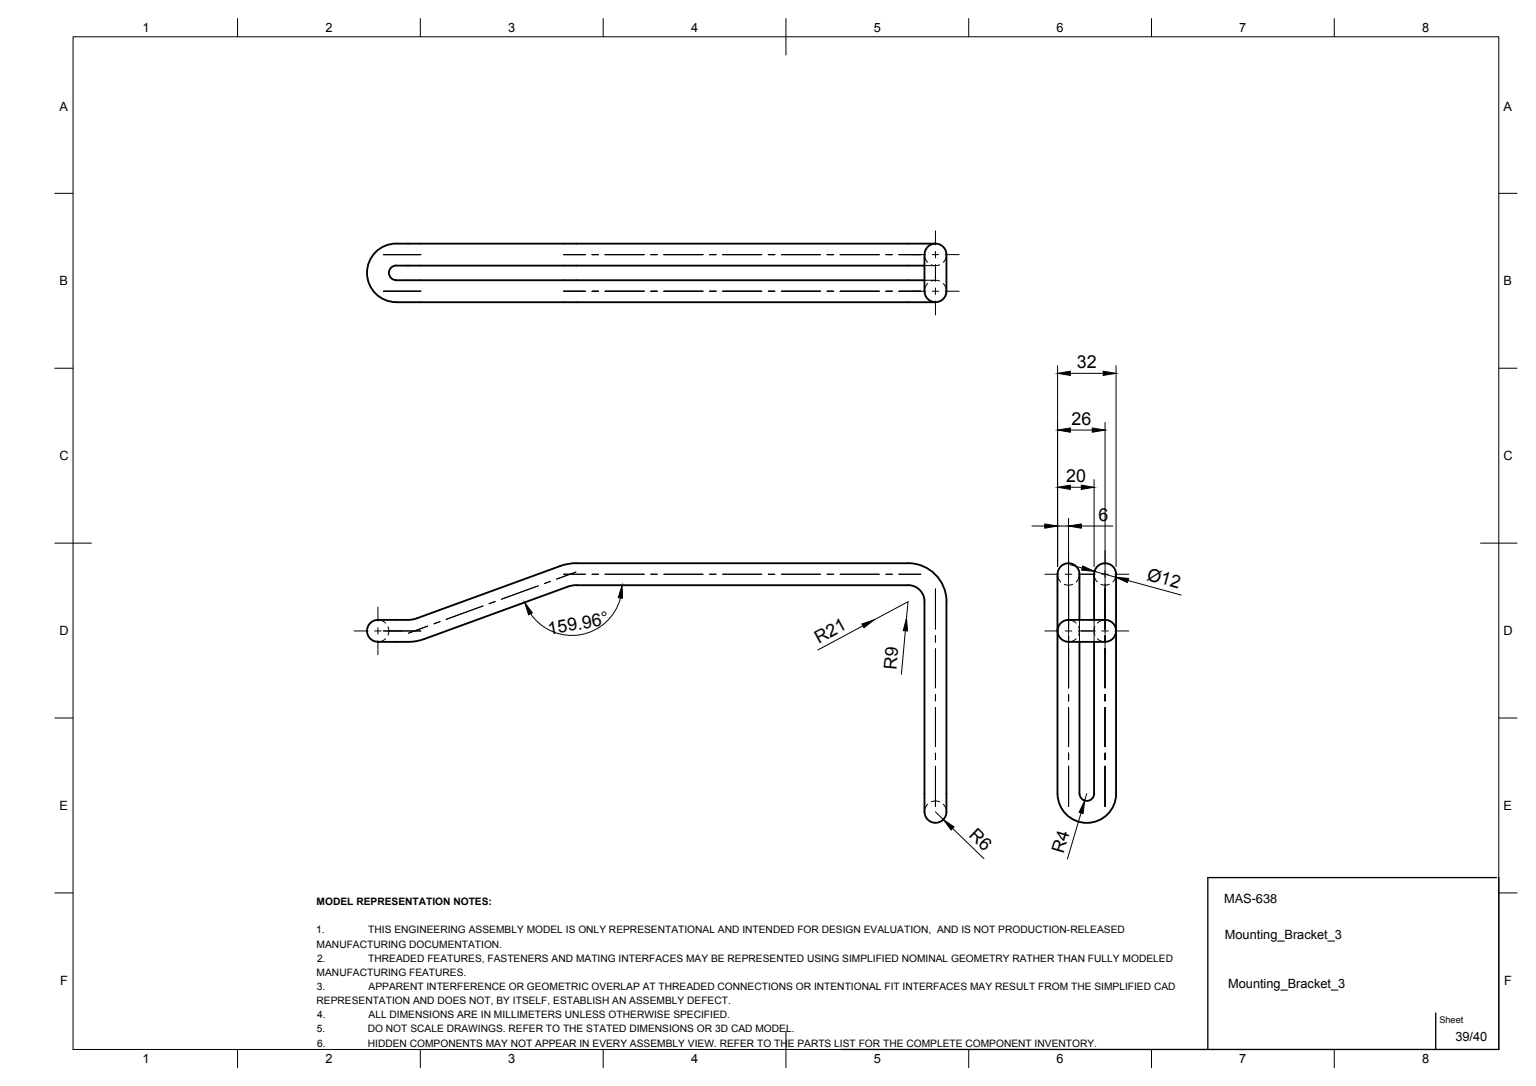
ISO-10303-21;
HEADER;
FILE_DESCRIPTION((''),'2;1');
FILE_NAME('Mounting_Bracket_3.step','2026-10-09T12:00:21-07:00',(''),(''),'','','');
FILE_SCHEMA (('AUTOMOTIVE_DESIGN { 1 0 10303 214 3 1 1 }'));
ENDSEC;
DATA;
#10=MECHANICAL_DESIGN_GEOMETRIC_PRESENTATION_REPRESENTATION('',(#434),#10334);
#176=CYLINDRICAL_SURFACE('',#4377,0.600000000000001) ;
#177=CYLINDRICAL_SURFACE('',#4378,0.600000000000001) ;
#178=CYLINDRICAL_SURFACE('',#4379,0.599999999999997) ;
#179=CYLINDRICAL_SURFACE('',#4380,0.600000000000001) ;
#180=CYLINDRICAL_SURFACE('',#4381,0.600000000000001) ;
#181=CYLINDRICAL_SURFACE('',#4382,0.600000000000001) ;
#182=CYLINDRICAL_SURFACE('',#4383,0.599999999999997) ;
#183=CYLINDRICAL_SURFACE('',#4384,0.600000000000001) ;
#362=SHAPE_REPRESENTATION_RELATIONSHIP('SRR','None',#10480,#394) ;
#394=ADVANCED_BREP_SHAPE_REPRESENTATION('',(#466),#10332) ;
#434=STYLED_ITEM('',(#10631),#466) ;
#466=MANIFOLD_SOLID_BREP('Body1',#3588) ;
#674=LINE('',#10153,#832) ;
#675=LINE('',#10155,#833) ;
#676=LINE('',#10157,#834) ;
#677=LINE('',#10159,#835) ;
#678=LINE('',#10161,#836) ;
#679=LINE('',#10163,#837) ;
#680=LINE('',#10165,#838) ;
#681=LINE('',#10167,#839) ;
#832=VECTOR('',#5456,0.600000000000001) ;
#833=VECTOR('',#5459,0.600000000000001) ;
#834=VECTOR('',#5462,0.599999999999997) ;
#835=VECTOR('',#5465,0.600000000000001) ;
#836=VECTOR('',#5468,0.600000000000001) ;
#837=VECTOR('',#5471,0.600000000000001) ;
#838=VECTOR('',#5474,0.599999999999997) ;
#839=VECTOR('',#5477,0.600000000000001) ;
#1018=FACE_OUTER_BOUND('',#1226,.T.) ;
#1019=FACE_OUTER_BOUND('',#1227,.T.) ;
#1020=FACE_OUTER_BOUND('',#1228,.T.) ;
#1021=FACE_OUTER_BOUND('',#1229,.T.) ;
#1022=FACE_OUTER_BOUND('',#1230,.T.) ;
#1023=FACE_OUTER_BOUND('',#1231,.T.) ;
#1024=FACE_OUTER_BOUND('',#1232,.T.) ;
#1025=FACE_OUTER_BOUND('',#1233,.T.) ;
#1026=FACE_OUTER_BOUND('',#1234,.T.) ;
#1027=FACE_OUTER_BOUND('',#1235,.T.) ;
#1028=FACE_OUTER_BOUND('',#1236,.T.) ;
#1029=FACE_OUTER_BOUND('',#1237,.T.) ;
#1030=FACE_OUTER_BOUND('',#1238,.T.) ;
#1031=FACE_OUTER_BOUND('',#1239,.T.) ;
#1032=FACE_OUTER_BOUND('',#1240,.T.) ;
#1033=FACE_OUTER_BOUND('',#1241,.T.) ;
#1226=EDGE_LOOP('',(#3133,#3134,#3135,#3136,#3137)) ;
#1227=EDGE_LOOP('',(#3138,#3139,#3140,#3141)) ;
#1228=EDGE_LOOP('',(#3142,#3143,#3144,#3145,#3146,#3147)) ;
#1229=EDGE_LOOP('',(#3148,#3149,#3150,#3151,#3152,#3153)) ;
#1230=EDGE_LOOP('',(#3154,#3155,#3156,#3157,#3158,#3159)) ;
#1231=EDGE_LOOP('',(#3160,#3161,#3162,#3163,#3164)) ;
#1232=EDGE_LOOP('',(#3165,#3166,#3167,#3168)) ;
#1233=EDGE_LOOP('',(#3169,#3170,#3171,#3172,#3173,#3174)) ;
#1234=EDGE_LOOP('',(#3175,#3176,#3177,#3178,#3179,#3180)) ;
#1235=EDGE_LOOP('',(#3181,#3182,#3183,#3184)) ;
#1236=EDGE_LOOP('',(#3185,#3186,#3187,#3188,#3189)) ;
#1237=EDGE_LOOP('',(#3190,#3191,#3192,#3193,#3194,#3195)) ;
#1238=EDGE_LOOP('',(#3196,#3197,#3198,#3199,#3200,#3201)) ;
#1239=EDGE_LOOP('',(#3202,#3203,#3204,#3205)) ;
#1240=EDGE_LOOP('',(#3206,#3207,#3208,#3209,#3210)) ;
#1241=EDGE_LOOP('',(#3211,#3212,#3213,#3214,#3215,#3216)) ;
#1431=CIRCLE('',#4336,0.600000000000001) ;
#1432=CIRCLE('',#4337,0.9) ;
#1433=CIRCLE('',#4338,0.600000000000001) ;
#1434=CIRCLE('',#4339,0.600000000000001) ;
#1435=CIRCLE('',#4341,0.600000000000001) ;
#1436=CIRCLE('',#4342,1.4) ;
#1437=CIRCLE('',#4343,0.600000000000001) ;
#1438=CIRCLE('',#4345,0.600000000000001) ;
#1439=CIRCLE('',#4346,0.600000000000001) ;
#1440=CIRCLE('',#4347,1.4) ;
#1441=CIRCLE('',#4348,0.600000000000001) ;
#1442=CIRCLE('',#4349,0.600000000000001) ;
#1443=CIRCLE('',#4351,0.600000000000001) ;
#1444=CIRCLE('',#4352,0.400000000000006) ;
#1445=CIRCLE('',#4353,0.600000000000001) ;
#1446=CIRCLE('',#4354,0.600000000000001) ;
#1447=CIRCLE('',#4355,0.600000000000001) ;
#1448=CIRCLE('',#4357,0.600000000000001) ;
#1449=CIRCLE('',#4358,0.600000000000001) ;
#1450=CIRCLE('',#4359,0.400000000000006) ;
#1451=CIRCLE('',#4360,0.600000000000001) ;
#1452=CIRCLE('',#4361,0.600000000000001) ;
#1453=CIRCLE('',#4363,0.600000000000001) ;
#1454=CIRCLE('',#4364,0.600000000000001) ;
#1455=CIRCLE('',#4365,0.9) ;
#1456=CIRCLE('',#4366,0.600000000000001) ;
#1457=CIRCLE('',#4368,0.600000000000001) ;
#1458=CIRCLE('',#4369,1.4) ;
#1459=CIRCLE('',#4370,0.600000000000001) ;
#1460=CIRCLE('',#4372,0.600000000000001) ;
#1461=CIRCLE('',#4373,0.600000000000001) ;
#1462=CIRCLE('',#4374,1.4) ;
#1463=CIRCLE('',#4375,0.600000000000001) ;
#1464=CIRCLE('',#4376,0.600000000000001) ;
#1758=VERTEX_POINT('',#10085) ;
#1759=VERTEX_POINT('',#10087) ;
#1760=VERTEX_POINT('',#10089) ;
#1761=VERTEX_POINT('',#10093) ;
#1762=VERTEX_POINT('',#10095) ;
#1763=VERTEX_POINT('',#10099) ;
#1764=VERTEX_POINT('',#10100) ;
#1765=VERTEX_POINT('',#10103) ;
#1766=VERTEX_POINT('',#10105) ;
#1767=VERTEX_POINT('',#10109) ;
#1768=VERTEX_POINT('',#10110) ;
#1769=VERTEX_POINT('',#10112) ;
#1770=VERTEX_POINT('',#10114) ;
#1771=VERTEX_POINT('',#10119) ;
#1772=VERTEX_POINT('',#10120) ;
#1773=VERTEX_POINT('',#10123) ;
#1774=VERTEX_POINT('',#10125) ;
#1775=VERTEX_POINT('',#10129) ;
#1776=VERTEX_POINT('',#10130) ;
#1777=VERTEX_POINT('',#10133) ;
#1778=VERTEX_POINT('',#10137) ;
#1779=VERTEX_POINT('',#10139) ;
#1780=VERTEX_POINT('',#10143) ;
#1781=VERTEX_POINT('',#10144) ;
#1782=VERTEX_POINT('',#10147) ;
#1783=VERTEX_POINT('',#10149) ;
#2223=EDGE_CURVE('',#1758,#1758,#1431,.T.) ;
#2224=EDGE_CURVE('',#1758,#1759,#1432,.T.) ;
#2225=EDGE_CURVE('',#1759,#1760,#1433,.T.) ;
#2226=EDGE_CURVE('',#1760,#1759,#1434,.T.) ;
#2227=EDGE_CURVE('',#1761,#1761,#1435,.T.) ;
#2228=EDGE_CURVE('',#1761,#1762,#1436,.T.) ;
#2229=EDGE_CURVE('',#1762,#1762,#1437,.T.) ;
#2230=EDGE_CURVE('',#1763,#1764,#1438,.T.) ;
#2231=EDGE_CURVE('',#1764,#1763,#1439,.T.) ;
#2232=EDGE_CURVE('',#1764,#1765,#1440,.T.) ;
#2233=EDGE_CURVE('',#1765,#1766,#1441,.T.) ;
#2234=EDGE_CURVE('',#1766,#1765,#1442,.T.) ;
#2235=EDGE_CURVE('',#1767,#1768,#1443,.T.) ;
#2236=EDGE_CURVE('',#1768,#1769,#1444,.T.) ;
#2237=EDGE_CURVE('',#1770,#1769,#1445,.T.) ;
#2238=EDGE_CURVE('',#1769,#1770,#1446,.T.) ;
#2239=EDGE_CURVE('',#1768,#1767,#1447,.T.) ;
#2240=EDGE_CURVE('',#1771,#1772,#1448,.T.) ;
#2241=EDGE_CURVE('',#1772,#1771,#1449,.T.) ;
#2242=EDGE_CURVE('',#1772,#1773,#1450,.T.) ;
#2243=EDGE_CURVE('',#1773,#1774,#1451,.T.) ;
#2244=EDGE_CURVE('',#1774,#1773,#1452,.T.) ;
#2245=EDGE_CURVE('',#1775,#1776,#1453,.T.) ;
#2246=EDGE_CURVE('',#1776,#1775,#1454,.T.) ;
#2247=EDGE_CURVE('',#1776,#1777,#1455,.T.) ;
#2248=EDGE_CURVE('',#1777,#1777,#1456,.T.) ;
#2249=EDGE_CURVE('',#1778,#1778,#1457,.T.) ;
#2250=EDGE_CURVE('',#1778,#1779,#1458,.T.) ;
#2251=EDGE_CURVE('',#1779,#1779,#1459,.T.) ;
#2252=EDGE_CURVE('',#1780,#1781,#1460,.T.) ;
#2253=EDGE_CURVE('',#1781,#1780,#1461,.T.) ;
#2254=EDGE_CURVE('',#1781,#1782,#1462,.T.) ;
#2255=EDGE_CURVE('',#1782,#1783,#1463,.T.) ;
#2256=EDGE_CURVE('',#1783,#1782,#1464,.T.) ;
#2257=EDGE_CURVE('',#1771,#1760,#674,.T.) ;
#2258=EDGE_CURVE('',#1758,#1762,#675,.T.) ;
#2259=EDGE_CURVE('',#1761,#1766,#676,.T.) ;
#2260=EDGE_CURVE('',#1763,#1767,#677,.T.) ;
#2261=EDGE_CURVE('',#1774,#1775,#678,.T.) ;
#2262=EDGE_CURVE('',#1777,#1778,#679,.T.) ;
#2263=EDGE_CURVE('',#1779,#1780,#680,.T.) ;
#2264=EDGE_CURVE('',#1783,#1770,#681,.T.) ;
#3133=ORIENTED_EDGE('',*,*,#2223,.F.) ;
#3134=ORIENTED_EDGE('',*,*,#2224,.T.) ;
#3135=ORIENTED_EDGE('',*,*,#2225,.T.) ;
#3136=ORIENTED_EDGE('',*,*,#2226,.T.) ;
#3137=ORIENTED_EDGE('',*,*,#2224,.F.) ;
#3138=ORIENTED_EDGE('',*,*,#2227,.F.) ;
#3139=ORIENTED_EDGE('',*,*,#2228,.T.) ;
#3140=ORIENTED_EDGE('',*,*,#2229,.T.) ;
#3141=ORIENTED_EDGE('',*,*,#2228,.F.) ;
#3142=ORIENTED_EDGE('',*,*,#2230,.F.) ;
#3143=ORIENTED_EDGE('',*,*,#2231,.F.) ;
#3144=ORIENTED_EDGE('',*,*,#2232,.T.) ;
#3145=ORIENTED_EDGE('',*,*,#2233,.T.) ;
#3146=ORIENTED_EDGE('',*,*,#2234,.T.) ;
#3147=ORIENTED_EDGE('',*,*,#2232,.F.) ;
#3148=ORIENTED_EDGE('',*,*,#2235,.T.) ;
#3149=ORIENTED_EDGE('',*,*,#2236,.T.) ;
#3150=ORIENTED_EDGE('',*,*,#2237,.F.) ;
#3151=ORIENTED_EDGE('',*,*,#2238,.F.) ;
#3152=ORIENTED_EDGE('',*,*,#2236,.F.) ;
#3153=ORIENTED_EDGE('',*,*,#2239,.T.) ;
#3154=ORIENTED_EDGE('',*,*,#2240,.F.) ;
#3155=ORIENTED_EDGE('',*,*,#2241,.F.) ;
#3156=ORIENTED_EDGE('',*,*,#2242,.T.) ;
#3157=ORIENTED_EDGE('',*,*,#2243,.T.) ;
#3158=ORIENTED_EDGE('',*,*,#2244,.T.) ;
#3159=ORIENTED_EDGE('',*,*,#2242,.F.) ;
#3160=ORIENTED_EDGE('',*,*,#2245,.F.) ;
#3161=ORIENTED_EDGE('',*,*,#2246,.F.) ;
#3162=ORIENTED_EDGE('',*,*,#2247,.T.) ;
#3163=ORIENTED_EDGE('',*,*,#2248,.T.) ;
#3164=ORIENTED_EDGE('',*,*,#2247,.F.) ;
#3165=ORIENTED_EDGE('',*,*,#2249,.F.) ;
#3166=ORIENTED_EDGE('',*,*,#2250,.T.) ;
#3167=ORIENTED_EDGE('',*,*,#2251,.T.) ;
#3168=ORIENTED_EDGE('',*,*,#2250,.F.) ;
#3169=ORIENTED_EDGE('',*,*,#2252,.F.) ;
#3170=ORIENTED_EDGE('',*,*,#2253,.F.) ;
#3171=ORIENTED_EDGE('',*,*,#2254,.T.) ;
#3172=ORIENTED_EDGE('',*,*,#2255,.T.) ;
#3173=ORIENTED_EDGE('',*,*,#2256,.T.) ;
#3174=ORIENTED_EDGE('',*,*,#2254,.F.) ;
#3175=ORIENTED_EDGE('',*,*,#2240,.T.) ;
#3176=ORIENTED_EDGE('',*,*,#2241,.T.) ;
#3177=ORIENTED_EDGE('',*,*,#2257,.T.) ;
#3178=ORIENTED_EDGE('',*,*,#2225,.F.) ;
#3179=ORIENTED_EDGE('',*,*,#2226,.F.) ;
#3180=ORIENTED_EDGE('',*,*,#2257,.F.) ;
#3181=ORIENTED_EDGE('',*,*,#2223,.T.) ;
#3182=ORIENTED_EDGE('',*,*,#2258,.T.) ;
#3183=ORIENTED_EDGE('',*,*,#2229,.F.) ;
#3184=ORIENTED_EDGE('',*,*,#2258,.F.) ;
#3185=ORIENTED_EDGE('',*,*,#2227,.T.) ;
#3186=ORIENTED_EDGE('',*,*,#2259,.T.) ;
#3187=ORIENTED_EDGE('',*,*,#2233,.F.) ;
#3188=ORIENTED_EDGE('',*,*,#2234,.F.) ;
#3189=ORIENTED_EDGE('',*,*,#2259,.F.) ;
#3190=ORIENTED_EDGE('',*,*,#2230,.T.) ;
#3191=ORIENTED_EDGE('',*,*,#2231,.T.) ;
#3192=ORIENTED_EDGE('',*,*,#2260,.T.) ;
#3193=ORIENTED_EDGE('',*,*,#2239,.F.) ;
#3194=ORIENTED_EDGE('',*,*,#2235,.F.) ;
#3195=ORIENTED_EDGE('',*,*,#2260,.F.) ;
#3196=ORIENTED_EDGE('',*,*,#2244,.F.) ;
#3197=ORIENTED_EDGE('',*,*,#2261,.T.) ;
#3198=ORIENTED_EDGE('',*,*,#2245,.T.) ;
#3199=ORIENTED_EDGE('',*,*,#2246,.T.) ;
#3200=ORIENTED_EDGE('',*,*,#2261,.F.) ;
#3201=ORIENTED_EDGE('',*,*,#2243,.F.) ;
#3202=ORIENTED_EDGE('',*,*,#2248,.F.) ;
#3203=ORIENTED_EDGE('',*,*,#2262,.T.) ;
#3204=ORIENTED_EDGE('',*,*,#2249,.T.) ;
#3205=ORIENTED_EDGE('',*,*,#2262,.F.) ;
#3206=ORIENTED_EDGE('',*,*,#2251,.F.) ;
#3207=ORIENTED_EDGE('',*,*,#2263,.T.) ;
#3208=ORIENTED_EDGE('',*,*,#2252,.T.) ;
#3209=ORIENTED_EDGE('',*,*,#2253,.T.) ;
#3210=ORIENTED_EDGE('',*,*,#2263,.F.) ;
#3211=ORIENTED_EDGE('',*,*,#2256,.F.) ;
#3212=ORIENTED_EDGE('',*,*,#2264,.T.) ;
#3213=ORIENTED_EDGE('',*,*,#2237,.T.) ;
#3214=ORIENTED_EDGE('',*,*,#2238,.T.) ;
#3215=ORIENTED_EDGE('',*,*,#2264,.F.) ;
#3216=ORIENTED_EDGE('',*,*,#2255,.F.) ;
#3343=TOROIDAL_SURFACE('',#4335,1.5,0.6) ;
#3344=TOROIDAL_SURFACE('',#4340,2.,0.6) ;
#3345=TOROIDAL_SURFACE('',#4344,2.,0.6) ;
#3346=TOROIDAL_SURFACE('',#4350,1.,0.6) ;
#3347=TOROIDAL_SURFACE('',#4356,1.,0.599999999999999) ;
#3348=TOROIDAL_SURFACE('',#4362,1.5,0.6) ;
#3349=TOROIDAL_SURFACE('',#4367,2.,0.6) ;
#3350=TOROIDAL_SURFACE('',#4371,2.,0.6) ;
#3526=ADVANCED_FACE('',(#1018),#3343,.T.) ;
#3527=ADVANCED_FACE('',(#1019),#3344,.T.) ;
#3528=ADVANCED_FACE('',(#1020),#3345,.T.) ;
#3529=ADVANCED_FACE('',(#1021),#3346,.T.) ;
#3530=ADVANCED_FACE('',(#1022),#3347,.T.) ;
#3531=ADVANCED_FACE('',(#1023),#3348,.T.) ;
#3532=ADVANCED_FACE('',(#1024),#3349,.T.) ;
#3533=ADVANCED_FACE('',(#1025),#3350,.T.) ;
#3534=ADVANCED_FACE('',(#1026),#176,.T.) ;
#3535=ADVANCED_FACE('',(#1027),#177,.T.) ;
#3536=ADVANCED_FACE('',(#1028),#178,.T.) ;
#3537=ADVANCED_FACE('',(#1029),#179,.T.) ;
#3538=ADVANCED_FACE('',(#1030),#180,.T.) ;
#3539=ADVANCED_FACE('',(#1031),#181,.T.) ;
#3540=ADVANCED_FACE('',(#1032),#182,.T.) ;
#3541=ADVANCED_FACE('',(#1033),#183,.T.) ;
#3588=CLOSED_SHELL('',(#3526,#3527,#3528,#3529,#3530,#3531,#3532,#3533,
#3534,#3535,#3536,#3537,#3538,#3539,#3540,#3541)) ;
#4334=AXIS2_PLACEMENT_3D('',#10083,#5368,#5369) ;
#4335=AXIS2_PLACEMENT_3D('',#10084,#5370,#5371) ;
#4336=AXIS2_PLACEMENT_3D('',#10086,#5372,#5373) ;
#4337=AXIS2_PLACEMENT_3D('',#10088,#5374,#5375) ;
#4338=AXIS2_PLACEMENT_3D('',#10090,#5376,#5377) ;
#4339=AXIS2_PLACEMENT_3D('',#10091,#5378,#5379) ;
#4340=AXIS2_PLACEMENT_3D('',#10092,#5380,#5381) ;
#4341=AXIS2_PLACEMENT_3D('',#10094,#5382,#5383) ;
#4342=AXIS2_PLACEMENT_3D('',#10096,#5384,#5385) ;
#4343=AXIS2_PLACEMENT_3D('',#10097,#5386,#5387) ;
#4344=AXIS2_PLACEMENT_3D('',#10098,#5388,#5389) ;
#4345=AXIS2_PLACEMENT_3D('',#10101,#5390,#5391) ;
#4346=AXIS2_PLACEMENT_3D('',#10102,#5392,#5393) ;
#4347=AXIS2_PLACEMENT_3D('',#10104,#5394,#5395) ;
#4348=AXIS2_PLACEMENT_3D('',#10106,#5396,#5397) ;
#4349=AXIS2_PLACEMENT_3D('',#10107,#5398,#5399) ;
#4350=AXIS2_PLACEMENT_3D('',#10108,#5400,#5401) ;
#4351=AXIS2_PLACEMENT_3D('',#10111,#5402,#5403) ;
#4352=AXIS2_PLACEMENT_3D('',#10113,#5404,#5405) ;
#4353=AXIS2_PLACEMENT_3D('',#10115,#5406,#5407) ;
#4354=AXIS2_PLACEMENT_3D('',#10116,#5408,#5409) ;
#4355=AXIS2_PLACEMENT_3D('',#10117,#5410,#5411) ;
#4356=AXIS2_PLACEMENT_3D('',#10118,#5412,#5413) ;
#4357=AXIS2_PLACEMENT_3D('',#10121,#5414,#5415) ;
#4358=AXIS2_PLACEMENT_3D('',#10122,#5416,#5417) ;
#4359=AXIS2_PLACEMENT_3D('',#10124,#5418,#5419) ;
#4360=AXIS2_PLACEMENT_3D('',#10126,#5420,#5421) ;
#4361=AXIS2_PLACEMENT_3D('',#10127,#5422,#5423) ;
#4362=AXIS2_PLACEMENT_3D('',#10128,#5424,#5425) ;
#4363=AXIS2_PLACEMENT_3D('',#10131,#5426,#5427) ;
#4364=AXIS2_PLACEMENT_3D('',#10132,#5428,#5429) ;
#4365=AXIS2_PLACEMENT_3D('',#10134,#5430,#5431) ;
#4366=AXIS2_PLACEMENT_3D('',#10135,#5432,#5433) ;
#4367=AXIS2_PLACEMENT_3D('',#10136,#5434,#5435) ;
#4368=AXIS2_PLACEMENT_3D('',#10138,#5436,#5437) ;
#4369=AXIS2_PLACEMENT_3D('',#10140,#5438,#5439) ;
#4370=AXIS2_PLACEMENT_3D('',#10141,#5440,#5441) ;
#4371=AXIS2_PLACEMENT_3D('',#10142,#5442,#5443) ;
#4372=AXIS2_PLACEMENT_3D('',#10145,#5444,#5445) ;
#4373=AXIS2_PLACEMENT_3D('',#10146,#5446,#5447) ;
#4374=AXIS2_PLACEMENT_3D('',#10148,#5448,#5449) ;
#4375=AXIS2_PLACEMENT_3D('',#10150,#5450,#5451) ;
#4376=AXIS2_PLACEMENT_3D('',#10151,#5452,#5453) ;
#4377=AXIS2_PLACEMENT_3D('',#10152,#5454,#5455) ;
#4378=AXIS2_PLACEMENT_3D('',#10154,#5457,#5458) ;
#4379=AXIS2_PLACEMENT_3D('',#10156,#5460,#5461) ;
#4380=AXIS2_PLACEMENT_3D('',#10158,#5463,#5464) ;
#4381=AXIS2_PLACEMENT_3D('',#10160,#5466,#5467) ;
#4382=AXIS2_PLACEMENT_3D('',#10162,#5469,#5470) ;
#4383=AXIS2_PLACEMENT_3D('',#10164,#5472,#5473) ;
#4384=AXIS2_PLACEMENT_3D('',#10166,#5475,#5476) ;
#5368=DIRECTION('axis',(0.,0.,1.)) ;
#5369=DIRECTION('refdir',(1.,0.,0.)) ;
#5370=DIRECTION('center_axis',(6.88094734232038E-15,0.,-1.)) ;
#5371=DIRECTION('ref_axis',(1.,0.,6.76707367390572E-15)) ;
#5372=DIRECTION('center_axis',(1.,0.,6.88094734232038E-15)) ;
#5373=DIRECTION('ref_axis',(6.88094734232038E-15,0.,-1.)) ;
#5374=DIRECTION('center_axis',(-6.88094734232038E-15,0.,1.)) ;
#5375=DIRECTION('ref_axis',(1.,0.,6.88094734232038E-15)) ;
#5376=DIRECTION('center_axis',(0.,1.,0.)) ;
#5377=DIRECTION('ref_axis',(4.62592926927148E-15,0.,-1.)) ;
#5378=DIRECTION('center_axis',(0.,1.,0.)) ;
#5379=DIRECTION('ref_axis',(4.62592926927148E-15,0.,-1.)) ;
#5380=DIRECTION('center_axis',(6.88094734232038E-15,0.,-1.)) ;
#5381=DIRECTION('ref_axis',(1.,0.,5.46571335200077E-15)) ;
#5382=DIRECTION('center_axis',(0.93947030108257,-0.342630345100702,6.46444567142303E-15)) ;
#5383=DIRECTION('ref_axis',(6.88775001098455E-15,1.86524785953259E-17,-1.)) ;
#5384=DIRECTION('center_axis',(-6.88094734232038E-15,0.,1.)) ;
#5385=DIRECTION('ref_axis',(1.,0.,6.88094734232038E-15)) ;
#5386=DIRECTION('center_axis',(1.,0.,6.88094734232038E-15)) ;
#5387=DIRECTION('ref_axis',(6.88094734232038E-15,0.,-1.)) ;
#5388=DIRECTION('center_axis',(-6.88094734232038E-15,0.,1.)) ;
#5389=DIRECTION('ref_axis',(-1.,0.,-5.46571335200077E-15)) ;
#5390=DIRECTION('center_axis',(1.,0.,6.88094734232038E-15)) ;
#5391=DIRECTION('ref_axis',(6.88094734232038E-15,0.,-1.)) ;
#5392=DIRECTION('center_axis',(1.,0.,6.88094734232038E-15)) ;
#5393=DIRECTION('ref_axis',(6.88094734232038E-15,0.,-1.)) ;
#5394=DIRECTION('center_axis',(6.88094734232038E-15,0.,-1.)) ;
#5395=DIRECTION('ref_axis',(-1.,0.,-6.88094734232038E-15)) ;
#5396=DIRECTION('center_axis',(0.93947030108257,-0.342630345100702,6.46444567142303E-15)) ;
#5397=DIRECTION('ref_axis',(6.61621824774427E-15,-7.25870098031252E-16,
-1.)) ;
#5398=DIRECTION('center_axis',(0.93947030108257,-0.342630345100702,6.46444567142303E-15)) ;
#5399=DIRECTION('ref_axis',(6.61621824774427E-15,-7.25870098031252E-16,
-1.)) ;
#5400=DIRECTION('center_axis',(0.,-1.,0.)) ;
#5401=DIRECTION('ref_axis',(-6.66133814775096E-15,0.,1.)) ;
#5402=DIRECTION('center_axis',(1.,0.,6.88094734232038E-15)) ;
#5403=DIRECTION('ref_axis',(6.88094734232038E-15,0.,-1.)) ;
#5404=DIRECTION('center_axis',(0.,1.,0.)) ;
#5405=DIRECTION('ref_axis',(-8.88178419700113E-15,0.,1.)) ;
#5406=DIRECTION('center_axis',(-1.,0.,-6.98296267768627E-15)) ;
#5407=DIRECTION('ref_axis',(-6.98296267768627E-15,0.,1.)) ;
#5408=DIRECTION('center_axis',(-1.,0.,-6.98296267768627E-15)) ;
#5409=DIRECTION('ref_axis',(-6.98296267768627E-15,0.,1.)) ;
#5410=DIRECTION('center_axis',(1.,0.,6.88094734232038E-15)) ;
#5411=DIRECTION('ref_axis',(6.88094734232038E-15,0.,-1.)) ;
#5412=DIRECTION('center_axis',(-1.,0.,-6.98296267768627E-15)) ;
#5413=DIRECTION('ref_axis',(-6.66133814775096E-15,0.,1.)) ;
#5414=DIRECTION('center_axis',(0.,1.,0.)) ;
#5415=DIRECTION('ref_axis',(4.62592926927148E-15,0.,-1.)) ;
#5416=DIRECTION('center_axis',(0.,1.,0.)) ;
#5417=DIRECTION('ref_axis',(4.62592926927148E-15,0.,-1.)) ;
#5418=DIRECTION('center_axis',(1.,0.,6.98296267768627E-15)) ;
#5419=DIRECTION('ref_axis',(-6.98296267768627E-15,0.,1.)) ;
#5420=DIRECTION('center_axis',(0.,-1.,0.)) ;
#5421=DIRECTION('ref_axis',(-9.25185853854296E-15,0.,1.)) ;
#5422=DIRECTION('center_axis',(0.,-1.,0.)) ;
#5423=DIRECTION('ref_axis',(-9.25185853854296E-15,0.,1.)) ;
#5424=DIRECTION('center_axis',(-6.98296267768627E-15,0.,1.)) ;
#5425=DIRECTION('ref_axis',(1.,0.,6.76707367390572E-15)) ;
#5426=DIRECTION('center_axis',(0.,-1.,0.)) ;
#5427=DIRECTION('ref_axis',(-9.25185853854296E-15,0.,1.)) ;
#5428=DIRECTION('center_axis',(0.,-1.,0.)) ;
#5429=DIRECTION('ref_axis',(-9.25185853854296E-15,0.,1.)) ;
#5430=DIRECTION('center_axis',(6.98296267768627E-15,0.,-1.)) ;
#5431=DIRECTION('ref_axis',(1.,0.,6.98296267768627E-15)) ;
#5432=DIRECTION('center_axis',(-1.,0.,-6.98296267768627E-15)) ;
#5433=DIRECTION('ref_axis',(-6.98296267768627E-15,0.,1.)) ;
#5434=DIRECTION('center_axis',(-6.98296267768627E-15,0.,1.)) ;
#5435=DIRECTION('ref_axis',(1.,0.,5.46571335200077E-15)) ;
#5436=DIRECTION('center_axis',(-1.,0.,-6.98296267768627E-15)) ;
#5437=DIRECTION('ref_axis',(-6.98296267768627E-15,0.,1.)) ;
#5438=DIRECTION('center_axis',(6.98296267768627E-15,0.,-1.)) ;
#5439=DIRECTION('ref_axis',(1.,0.,6.98296267768627E-15)) ;
#5440=DIRECTION('center_axis',(-0.93947030108257,0.342630345100702,-6.56028604925426E-15)) ;
#5441=DIRECTION('ref_axis',(-6.97778919960152E-15,1.41853431355683E-17,
1.)) ;
#5442=DIRECTION('center_axis',(6.98296267768627E-15,0.,-1.)) ;
#5443=DIRECTION('ref_axis',(-1.,0.,-5.46571335200077E-15)) ;
#5444=DIRECTION('center_axis',(-0.93947030108257,0.342630345100702,-6.56028604925426E-15)) ;
#5445=DIRECTION('ref_axis',(-7.24932096284181E-15,-7.30337233491011E-16,
1.)) ;
#5446=DIRECTION('center_axis',(-0.93947030108257,0.342630345100702,-6.56028604925426E-15)) ;
#5447=DIRECTION('ref_axis',(-7.24932096284181E-15,-7.30337233491011E-16,
1.)) ;
#5448=DIRECTION('center_axis',(-6.98296267768627E-15,0.,1.)) ;
#5449=DIRECTION('ref_axis',(-1.,0.,-6.98296267768627E-15)) ;
#5450=DIRECTION('center_axis',(-1.,0.,-6.98296267768627E-15)) ;
#5451=DIRECTION('ref_axis',(-6.98296267768627E-15,0.,1.)) ;
#5452=DIRECTION('center_axis',(-1.,0.,-6.98296267768627E-15)) ;
#5453=DIRECTION('ref_axis',(-6.98296267768627E-15,0.,1.)) ;
#5454=DIRECTION('center_axis',(0.,-1.,0.)) ;
#5455=DIRECTION('ref_axis',(4.62592926927148E-15,0.,-1.)) ;
#5456=DIRECTION('',(0.,1.,0.)) ;
#5457=DIRECTION('center_axis',(-1.,1.91189112624469E-17,-6.88094734232038E-15)) ;
#5458=DIRECTION('ref_axis',(1.91189112624469E-17,1.,1.31556221639393E-31)) ;
#5459=DIRECTION('',(1.,-1.91189112624469E-17,6.88094734232038E-15)) ;
#5460=DIRECTION('center_axis',(-0.93947030108257,0.342630345100702,-6.46444567142303E-15)) ;
#5461=DIRECTION('ref_axis',(0.342630345100702,0.93947030108257,-2.26638564151121E-29)) ;
#5462=DIRECTION('',(0.93947030108257,-0.342630345100702,6.46444567142303E-15)) ;
#5463=DIRECTION('center_axis',(-1.,0.,-6.88094734232038E-15)) ;
#5464=DIRECTION('ref_axis',(6.88094734232038E-15,0.,-1.)) ;
#5465=DIRECTION('',(1.,0.,6.88094734232038E-15)) ;
#5466=DIRECTION('center_axis',(0.,-1.,0.)) ;
#5467=DIRECTION('ref_axis',(-9.25185853854296E-15,0.,1.)) ;
#5468=DIRECTION('',(0.,1.,0.)) ;
#5469=DIRECTION('center_axis',(-1.,1.91189112624469E-17,-6.98296267768627E-15)) ;
#5470=DIRECTION('ref_axis',(1.91189112624469E-17,1.,1.33506643783662E-31)) ;
#5471=DIRECTION('',(1.,-1.91189112624469E-17,6.98296267768627E-15)) ;
#5472=DIRECTION('center_axis',(-0.93947030108257,0.342630345100702,-6.56028604925426E-15)) ;
#5473=DIRECTION('ref_axis',(0.342630345100702,0.93947030108257,-2.29769075252585E-29)) ;
#5474=DIRECTION('',(0.93947030108257,-0.342630345100702,6.56028604925426E-15)) ;
#5475=DIRECTION('center_axis',(-1.,0.,-6.98296267768627E-15)) ;
#5476=DIRECTION('ref_axis',(-6.98296267768627E-15,0.,1.)) ;
#5477=DIRECTION('',(1.,0.,6.98296267768627E-15)) ;
#10083=CARTESIAN_POINT('',(0.,0.,0.)) ;
#10084=CARTESIAN_POINT('Origin',(-11.7723119842408,67.0830586252741,69.2224337400006)) ;
#10085=CARTESIAN_POINT('',(-11.7723119842408,67.9830586252741,69.2224337400007)) ;
#10086=CARTESIAN_POINT('Origin',(-11.7723119842408,68.5830586252741,69.2224337400006)) ;
#10087=CARTESIAN_POINT('',(-12.6723119842408,67.0830586252741,69.2224337400006)) ;
#10088=CARTESIAN_POINT('Origin',(-11.7723119842408,67.0830586252741,69.2224337400006)) ;
#10089=CARTESIAN_POINT('',(-13.2723119842408,67.0830586252741,69.8224337400006)) ;
#10090=CARTESIAN_POINT('Origin',(-13.2723119842408,67.0830586252741,69.2224337400006)) ;
#10091=CARTESIAN_POINT('Origin',(-13.2723119842408,67.0830586252741,69.2224337400006)) ;
#10092=CARTESIAN_POINT('Origin',(6.37436438413731,66.5830586252741,69.2224337400008)) ;
#10093=CARTESIAN_POINT('',(6.85404686727829,67.8983170467897,69.2224337400008)) ;
#10094=CARTESIAN_POINT('Origin',(7.05962507433871,68.4619992274392,69.2224337400008)) ;
#10095=CARTESIAN_POINT('',(6.37436438413731,67.9830586252741,69.2224337400007)) ;
#10096=CARTESIAN_POINT('Origin',(6.37436438413731,66.5830586252741,69.2224337400008)) ;
#10097=CARTESIAN_POINT('Origin',(6.37436438413731,68.5830586252741,69.2224337400008)) ;
#10098=CARTESIAN_POINT('Origin',(15.5810116473812,67.4830586252741,69.2224337400008)) ;
#10099=CARTESIAN_POINT('',(15.5810116473812,65.4830586252741,69.8224337400008)) ;
#10100=CARTESIAN_POINT('',(15.5810116473812,66.0830586252741,69.2224337400008)) ;
#10101=CARTESIAN_POINT('Origin',(15.5810116473812,65.4830586252741,69.2224337400008)) ;
#10102=CARTESIAN_POINT('Origin',(15.5810116473812,65.4830586252741,69.2224337400008)) ;
#10103=CARTESIAN_POINT('',(15.1013291642402,66.1678002037585,69.2224337400008)) ;
#10104=CARTESIAN_POINT('Origin',(15.5810116473812,67.4830586252741,69.2224337400008)) ;
#10105=CARTESIAN_POINT('',(14.6901727501194,65.0404358424594,69.2224337400008)) ;
#10106=CARTESIAN_POINT('Origin',(14.8957509571798,65.604118023109,69.2224337400008)) ;
#10107=CARTESIAN_POINT('Origin',(14.8957509571798,65.604118023109,69.2224337400008)) ;
#10108=CARTESIAN_POINT('Origin',(16.2276880157593,65.4830586252741,68.2224337400008)) ;
#10109=CARTESIAN_POINT('',(16.2276880157592,65.4830586252741,69.8224337400008)) ;
#10110=CARTESIAN_POINT('',(16.2276880157593,65.4830586252741,68.6224337400008)) ;
#10111=CARTESIAN_POINT('Origin',(16.2276880157593,65.4830586252741,69.2224337400008)) ;
#10112=CARTESIAN_POINT('',(16.2276880157593,65.4830586252741,67.8224337400008)) ;
#10113=CARTESIAN_POINT('Origin',(16.2276880157593,65.4830586252741,68.2224337400008)) ;
#10114=CARTESIAN_POINT('',(16.2276880157593,65.4830586252741,66.6224337400008)) ;
#10115=CARTESIAN_POINT('Origin',(16.2276880157593,65.4830586252741,67.2224337400008)) ;
#10116=CARTESIAN_POINT('Origin',(16.2276880157593,65.4830586252741,67.2224337400008)) ;
#10117=CARTESIAN_POINT('Origin',(16.2276880157593,65.4830586252741,69.2224337400008)) ;
#10118=CARTESIAN_POINT('Origin',(-13.2723119842407,56.5830586252741,68.2224337400006)) ;
#10119=CARTESIAN_POINT('',(-13.2723119842408,56.5830586252741,69.8224337400006)) ;
#10120=CARTESIAN_POINT('',(-13.2723119842407,56.5830586252741,68.6224337400006)) ;
#10121=CARTESIAN_POINT('Origin',(-13.2723119842408,56.5830586252741,69.2224337400006)) ;
#10122=CARTESIAN_POINT('Origin',(-13.2723119842408,56.5830586252741,69.2224337400006)) ;
#10123=CARTESIAN_POINT('',(-13.2723119842407,56.5830586252741,67.8224337400006)) ;
#10124=CARTESIAN_POINT('Origin',(-13.2723119842407,56.5830586252741,68.2224337400006)) ;
#10125=CARTESIAN_POINT('',(-13.2723119842407,56.5830586252741,66.6224337400006)) ;
#10126=CARTESIAN_POINT('Origin',(-13.2723119842407,56.5830586252741,67.2224337400006)) ;
#10127=CARTESIAN_POINT('Origin',(-13.2723119842407,56.5830586252741,67.2224337400006)) ;
#10128=CARTESIAN_POINT('Origin',(-11.7723119842407,67.0830586252741,67.2224337400006)) ;
#10129=CARTESIAN_POINT('',(-13.2723119842407,67.0830586252741,66.6224337400006)) ;
#10130=CARTESIAN_POINT('',(-12.6723119842407,67.0830586252741,67.2224337400006)) ;
#10131=CARTESIAN_POINT('Origin',(-13.2723119842407,67.0830586252741,67.2224337400006)) ;
#10132=CARTESIAN_POINT('Origin',(-13.2723119842407,67.0830586252741,67.2224337400006)) ;
#10133=CARTESIAN_POINT('',(-11.7723119842407,67.9830586252741,67.2224337400007)) ;
#10134=CARTESIAN_POINT('Origin',(-11.7723119842407,67.0830586252741,67.2224337400006)) ;
#10135=CARTESIAN_POINT('Origin',(-11.7723119842407,68.5830586252741,67.2224337400006)) ;
#10136=CARTESIAN_POINT('Origin',(6.37436438413732,66.5830586252741,67.2224337400008)) ;
#10137=CARTESIAN_POINT('',(6.37436438413732,67.9830586252741,67.2224337400007)) ;
#10138=CARTESIAN_POINT('Origin',(6.37436438413732,68.5830586252741,67.2224337400008)) ;
#10139=CARTESIAN_POINT('',(6.8540468672783,67.8983170467897,67.2224337400008)) ;
#10140=CARTESIAN_POINT('Origin',(6.37436438413732,66.5830586252741,67.2224337400008)) ;
#10141=CARTESIAN_POINT('Origin',(7.05962507433873,68.4619992274392,67.2224337400008)) ;
#10142=CARTESIAN_POINT('Origin',(15.5810116473812,67.4830586252741,67.2224337400008)) ;
#10143=CARTESIAN_POINT('',(14.6901727501194,65.0404358424594,67.2224337400008)) ;
#10144=CARTESIAN_POINT('',(15.1013291642402,66.1678002037585,67.2224337400008)) ;
#10145=CARTESIAN_POINT('Origin',(14.8957509571798,65.604118023109,67.2224337400008)) ;
#10146=CARTESIAN_POINT('Origin',(14.8957509571798,65.604118023109,67.2224337400008)) ;
#10147=CARTESIAN_POINT('',(15.5810116473812,66.0830586252741,67.2224337400008)) ;
#10148=CARTESIAN_POINT('Origin',(15.5810116473812,67.4830586252741,67.2224337400008)) ;
#10149=CARTESIAN_POINT('',(15.5810116473812,65.4830586252741,66.6224337400008)) ;
#10150=CARTESIAN_POINT('Origin',(15.5810116473812,65.4830586252741,67.2224337400008)) ;
#10151=CARTESIAN_POINT('Origin',(15.5810116473812,65.4830586252741,67.2224337400008)) ;
#10152=CARTESIAN_POINT('Origin',(-13.2723119842408,67.0830586252741,69.2224337400006)) ;
#10153=CARTESIAN_POINT('',(-13.2723119842408,67.0830586252741,69.8224337400006)) ;
#10154=CARTESIAN_POINT('Origin',(6.37436438413731,68.5830586252741,69.2224337400008)) ;
#10155=CARTESIAN_POINT('',(6.37436438413731,67.9830586252741,69.2224337400008)) ;
#10156=CARTESIAN_POINT('Origin',(14.8957509571798,65.6041180231089,69.2224337400008)) ;
#10157=CARTESIAN_POINT('',(14.6901727501194,65.0404358424594,69.2224337400008)) ;
#10158=CARTESIAN_POINT('Origin',(16.2276880157593,65.4830586252741,69.2224337400008)) ;
#10159=CARTESIAN_POINT('',(16.2276880157593,65.4830586252741,69.8224337400008)) ;
#10160=CARTESIAN_POINT('Origin',(-13.2723119842407,67.0830586252741,67.2224337400006)) ;
#10161=CARTESIAN_POINT('',(-13.2723119842407,67.0830586252741,66.6224337400006)) ;
#10162=CARTESIAN_POINT('Origin',(6.37436438413732,68.5830586252741,67.2224337400008)) ;
#10163=CARTESIAN_POINT('',(6.37436438413732,67.9830586252741,67.2224337400008)) ;
#10164=CARTESIAN_POINT('Origin',(14.8957509571798,65.6041180231089,67.2224337400008)) ;
#10165=CARTESIAN_POINT('',(14.6901727501194,65.0404358424594,67.2224337400008)) ;
#10166=CARTESIAN_POINT('Origin',(16.2276880157593,65.4830586252741,67.2224337400008)) ;
#10167=CARTESIAN_POINT('',(16.2276880157593,65.4830586252741,66.6224337400008)) ;
#10295=UNCERTAINTY_MEASURE_WITH_UNIT(LENGTH_MEASURE(0.001),#10335,
'DISTANCE_ACCURACY_VALUE',
'Maximum model space distance between geometric entities at asserted c
onnectivities') ;
#10297=UNCERTAINTY_MEASURE_WITH_UNIT(LENGTH_MEASURE(0.001),#10335,
'DISTANCE_ACCURACY_VALUE',
'Maximum model space distance between geometric entities at asserted c
onnectivities') ;
#10332=(
GEOMETRIC_REPRESENTATION_CONTEXT(3)
GLOBAL_UNCERTAINTY_ASSIGNED_CONTEXT((#10295))
GLOBAL_UNIT_ASSIGNED_CONTEXT((#10335,#10337,#10338))
REPRESENTATION_CONTEXT('','3D')
) ;
#10334=(
GEOMETRIC_REPRESENTATION_CONTEXT(3)
GLOBAL_UNCERTAINTY_ASSIGNED_CONTEXT((#10297))
GLOBAL_UNIT_ASSIGNED_CONTEXT((#10335,#10337,#10338))
REPRESENTATION_CONTEXT('','3D')
) ;
#10335=(
LENGTH_UNIT()
NAMED_UNIT(*)
SI_UNIT(.CENTI.,.METRE.)
) ;
#10337=(
NAMED_UNIT(*)
PLANE_ANGLE_UNIT()
SI_UNIT($,.RADIAN.)
) ;
#10338=(
NAMED_UNIT(*)
SI_UNIT($,.STERADIAN.)
SOLID_ANGLE_UNIT()
) ;
#10373=SHAPE_DEFINITION_REPRESENTATION(#10436,#10480) ;
#10436=PRODUCT_DEFINITION_SHAPE('',$,#10517) ;
#10480=SHAPE_REPRESENTATION('',(#4334),#10332) ;
#10482=PRODUCT_DEFINITION_CONTEXT('part definition',#10592,'design') ;
#10517=PRODUCT_DEFINITION('Mounting_Bracket_3','Mounting_Bracket_3',#10553,
#10482) ;
#10553=PRODUCT_DEFINITION_FORMATION('',$,#10628) ;
#10592=APPLICATION_CONTEXT(
'Core Data for Automotive Mechanical Design Process') ;
#10593=PRODUCT_CONTEXT('part definition',#10592,'mechanical') ;
#10628=PRODUCT('Mounting_Bracket_3','Mounting_Bracket_3',$,(#10593)) ;
#10631=PRESENTATION_STYLE_ASSIGNMENT((#10635)) ;
#10635=SURFACE_STYLE_USAGE(.BOTH.,#10639) ;
#10639=SURFACE_SIDE_STYLE('',(#10643)) ;
#10643=SURFACE_STYLE_FILL_AREA(#10647) ;
#10647=FILL_AREA_STYLE('Opaque(25,25,25)',(#10651)) ;
#10651=FILL_AREA_STYLE_COLOUR('Opaque(25,25,25)',#10655) ;
#10655=COLOUR_RGB('Opaque(25,25,25)', 0.09019608, 0.27058824, 0.51372549) ;
ENDSEC;
END-ISO-10303-21;
